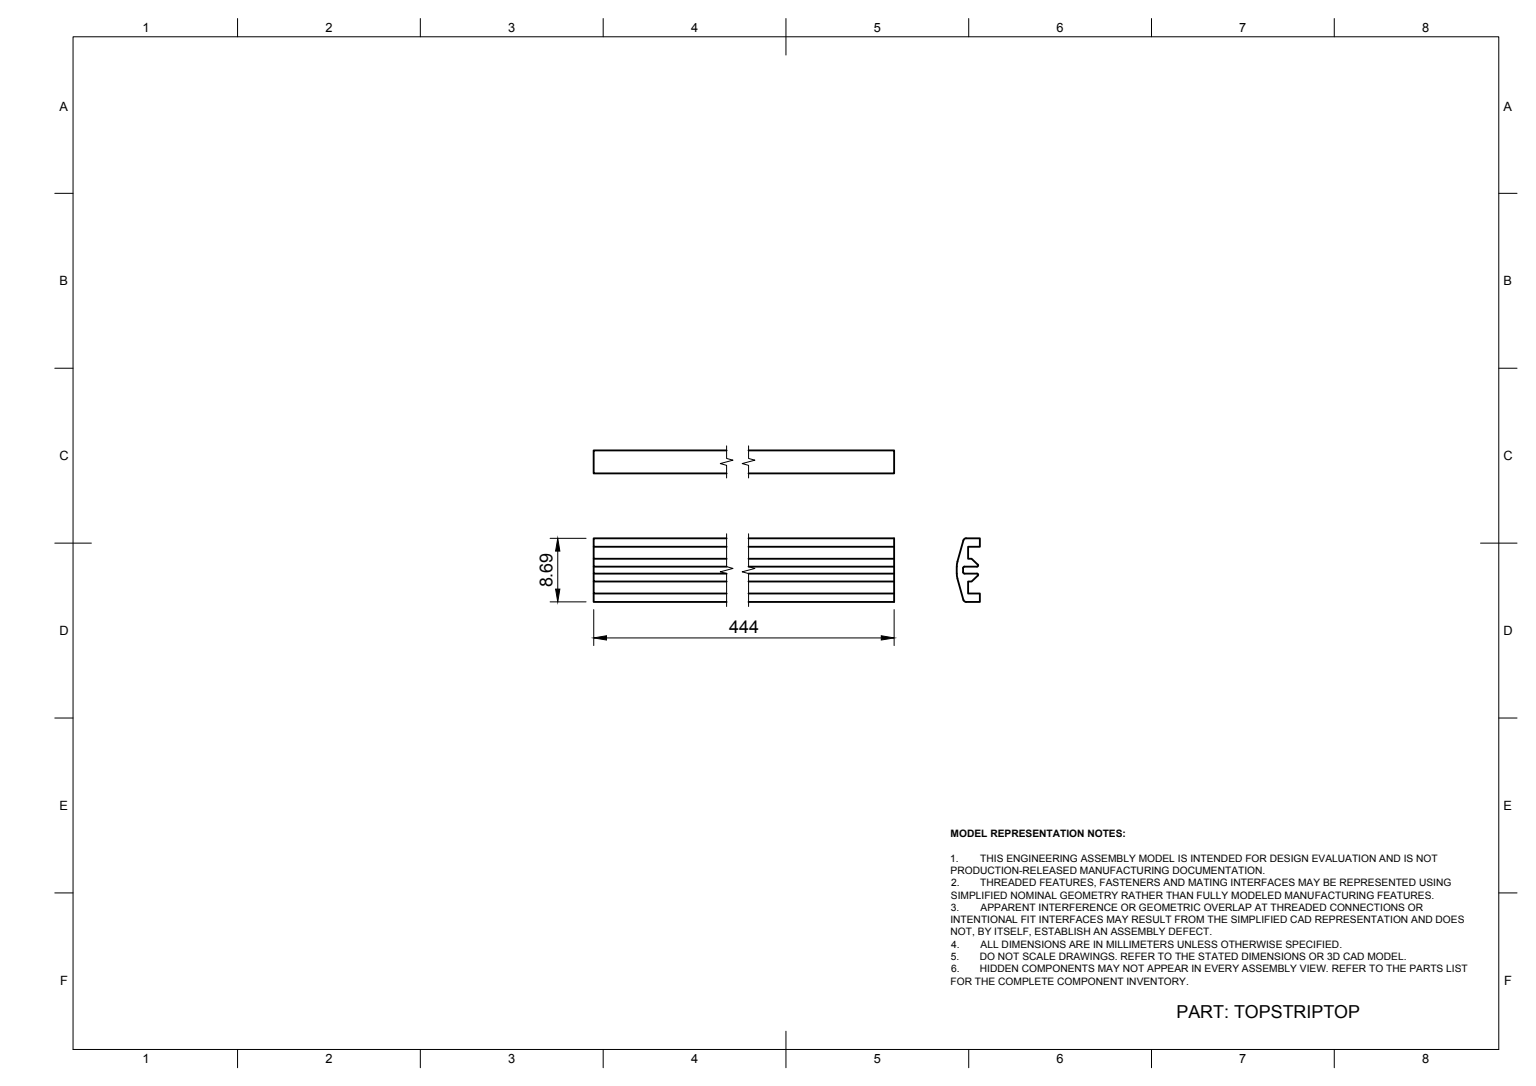
ISO-10303-21;
HEADER;
/* Generated by software containing ST-Developer
 * from STEP Tools, Inc. (www.steptools.com) 
 */

FILE_DESCRIPTION(
/* description */ (''),
/* implementation_level */ '2;1');

FILE_NAME(
/* name */ 'TopStripTop.step',
/* time_stamp */ '2026-10-05T11:01:41-07:00',
/* author */ (''),
/* organization */ (''),
/* preprocessor_version */ 'ST-DEVELOPER v20.2',
/* originating_system */ 'Autodesk Translation Framework v15.15.0.0',
/* authorisation */ '');

FILE_SCHEMA (('AUTOMOTIVE_DESIGN { 1 0 10303 214 3 1 1 }'));
ENDSEC;

DATA;
#10=MECHANICAL_DESIGN_GEOMETRIC_PRESENTATION_REPRESENTATION('',(#2138),#215609);
#2120=SHAPE_REPRESENTATION_RELATIONSHIP('SRR','None',#215645,#2129);
#2129=ADVANCED_BREP_SHAPE_REPRESENTATION('',(#2147),#215601);
#2138=STYLED_ITEM('',(#215698),#2147);
#2147=MANIFOLD_SOLID_BREP('Body1',#28081);
#2165=CYLINDRICAL_SURFACE('',#28237,0.203000000000002);
#2166=CYLINDRICAL_SURFACE('',#28240,0.203000000000002);
#2167=CYLINDRICAL_SURFACE('',#28243,0.159);
#2168=CYLINDRICAL_SURFACE('',#28251,0.381);
#2169=CYLINDRICAL_SURFACE('',#28254,2.54);
#2170=CYLINDRICAL_SURFACE('',#28257,2.54);
#2171=CYLINDRICAL_SURFACE('',#28260,0.381);
#2172=CYLINDRICAL_SURFACE('',#28268,0.159);
#2991=FACE_OUTER_BOUND('',#4304,.T.);
#2992=FACE_OUTER_BOUND('',#4305,.T.);
#2993=FACE_OUTER_BOUND('',#4306,.T.);
#2994=FACE_OUTER_BOUND('',#4307,.T.);
#2995=FACE_OUTER_BOUND('',#4308,.T.);
#2996=FACE_OUTER_BOUND('',#4309,.T.);
#2997=FACE_OUTER_BOUND('',#4310,.T.);
#2998=FACE_OUTER_BOUND('',#4311,.T.);
#2999=FACE_OUTER_BOUND('',#4312,.T.);
#3000=FACE_OUTER_BOUND('',#4313,.T.);
#3001=FACE_OUTER_BOUND('',#4314,.T.);
#3002=FACE_OUTER_BOUND('',#4315,.T.);
#3003=FACE_OUTER_BOUND('',#4316,.T.);
#3004=FACE_OUTER_BOUND('',#4317,.T.);
#3005=FACE_OUTER_BOUND('',#4318,.T.);
#3006=FACE_OUTER_BOUND('',#4319,.T.);
#3007=FACE_OUTER_BOUND('',#4320,.T.);
#3008=FACE_OUTER_BOUND('',#4321,.T.);
#3009=FACE_OUTER_BOUND('',#4322,.T.);
#3010=FACE_OUTER_BOUND('',#4323,.T.);
#3011=FACE_OUTER_BOUND('',#4324,.T.);
#3012=FACE_OUTER_BOUND('',#4325,.T.);
#3013=FACE_OUTER_BOUND('',#4326,.T.);
#3014=FACE_OUTER_BOUND('',#4327,.T.);
#3015=FACE_OUTER_BOUND('',#4328,.T.);
#3016=FACE_OUTER_BOUND('',#4329,.T.);
#3017=FACE_OUTER_BOUND('',#4330,.T.);
#3018=FACE_OUTER_BOUND('',#4331,.T.);
#4304=EDGE_LOOP('',(#17679,#17680,#17681,#17682,#17683,#17684,#17685,#17686,
#17687,#17688,#17689,#17690,#17691,#17692,#17693,#17694,#17695,#17696,#17697,
#17698,#17699,#17700,#17701,#17702,#17703,#17704));
#4305=EDGE_LOOP('',(#17705,#17706,#17707,#17708));
#4306=EDGE_LOOP('',(#17709,#17710,#17711,#17712));
#4307=EDGE_LOOP('',(#17713,#17714,#17715,#17716));
#4308=EDGE_LOOP('',(#17717,#17718,#17719,#17720));
#4309=EDGE_LOOP('',(#17721,#17722,#17723,#17724));
#4310=EDGE_LOOP('',(#17725,#17726,#17727,#17728));
#4311=EDGE_LOOP('',(#17729,#17730,#17731,#17732));
#4312=EDGE_LOOP('',(#17733,#17734,#17735,#17736));
#4313=EDGE_LOOP('',(#17737,#17738,#17739,#17740));
#4314=EDGE_LOOP('',(#17741,#17742,#17743,#17744));
#4315=EDGE_LOOP('',(#17745,#17746,#17747,#17748));
#4316=EDGE_LOOP('',(#17749,#17750,#17751,#17752));
#4317=EDGE_LOOP('',(#17753,#17754,#17755,#17756));
#4318=EDGE_LOOP('',(#17757,#17758,#17759,#17760));
#4319=EDGE_LOOP('',(#17761,#17762,#17763,#17764));
#4320=EDGE_LOOP('',(#17765,#17766,#17767,#17768));
#4321=EDGE_LOOP('',(#17769,#17770,#17771,#17772));
#4322=EDGE_LOOP('',(#17773,#17774,#17775,#17776));
#4323=EDGE_LOOP('',(#17777,#17778,#17779,#17780));
#4324=EDGE_LOOP('',(#17781,#17782,#17783,#17784));
#4325=EDGE_LOOP('',(#17785,#17786,#17787,#17788));
#4326=EDGE_LOOP('',(#17789,#17790,#17791,#17792));
#4327=EDGE_LOOP('',(#17793,#17794,#17795,#17796));
#4328=EDGE_LOOP('',(#17797,#17798,#17799,#17800));
#4329=EDGE_LOOP('',(#17801,#17802,#17803,#17804));
#4330=EDGE_LOOP('',(#17805,#17806,#17807,#17808));
#4331=EDGE_LOOP('',(#17809,#17810,#17811,#17812,#17813,#17814,#17815,#17816,
#17817,#17818,#17819,#17820,#17821,#17822,#17823,#17824,#17825,#17826,#17827,
#17828,#17829,#17830,#17831,#17832,#17833,#17834));
#5684=CIRCLE('',#28229,0.203000000000002);
#5685=CIRCLE('',#28230,0.203000000000002);
#5686=CIRCLE('',#28231,0.159);
#5687=CIRCLE('',#28232,0.381);
#5688=CIRCLE('',#28233,2.54);
#5689=CIRCLE('',#28234,2.54);
#5690=CIRCLE('',#28235,0.381);
#5691=CIRCLE('',#28236,0.159);
#5692=CIRCLE('',#28238,0.203000000000002);
#5693=CIRCLE('',#28241,0.203000000000002);
#5694=CIRCLE('',#28244,0.159);
#5695=CIRCLE('',#28252,0.381);
#5696=CIRCLE('',#28255,2.54);
#5697=CIRCLE('',#28258,2.54);
#5698=CIRCLE('',#28261,0.381);
#5699=CIRCLE('',#28269,0.159);
#6351=LINE('',#36139,#8196);
#6352=LINE('',#36143,#8197);
#6353=LINE('',#36147,#8198);
#6354=LINE('',#36151,#8199);
#6355=LINE('',#36153,#8200);
#6356=LINE('',#36155,#8201);
#6357=LINE('',#36157,#8202);
#6358=LINE('',#36159,#8203);
#6359=LINE('',#36161,#8204);
#6360=LINE('',#36165,#8205);
#6361=LINE('',#36169,#8206);
#6362=LINE('',#36173,#8207);
#6363=LINE('',#36177,#8208);
#6364=LINE('',#36179,#8209);
#6365=LINE('',#36181,#8210);
#6366=LINE('',#36183,#8211);
#6367=LINE('',#36185,#8212);
#6368=LINE('',#36187,#8213);
#6369=LINE('',#36191,#8214);
#6370=LINE('',#36194,#8215);
#6371=LINE('',#36197,#8216);
#6372=LINE('',#36198,#8217);
#6373=LINE('',#36202,#8218);
#6374=LINE('',#36205,#8219);
#6375=LINE('',#36206,#8220);
#6376=LINE('',#36210,#8221);
#6377=LINE('',#36213,#8222);
#6378=LINE('',#36214,#8223);
#6379=LINE('',#36217,#8224);
#6380=LINE('',#36218,#8225);
#6381=LINE('',#36221,#8226);
#6382=LINE('',#36222,#8227);
#6383=LINE('',#36225,#8228);
#6384=LINE('',#36226,#8229);
#6385=LINE('',#36229,#8230);
#6386=LINE('',#36230,#8231);
#6387=LINE('',#36233,#8232);
#6388=LINE('',#36234,#8233);
#6389=LINE('',#36238,#8234);
#6390=LINE('',#36241,#8235);
#6391=LINE('',#36242,#8236);
#6392=LINE('',#36246,#8237);
#6393=LINE('',#36249,#8238);
#6394=LINE('',#36250,#8239);
#6395=LINE('',#36254,#8240);
#6396=LINE('',#36257,#8241);
#6397=LINE('',#36258,#8242);
#6398=LINE('',#36262,#8243);
#6399=LINE('',#36265,#8244);
#6400=LINE('',#36266,#8245);
#6401=LINE('',#36269,#8246);
#6402=LINE('',#36270,#8247);
#6403=LINE('',#36273,#8248);
#6404=LINE('',#36274,#8249);
#6405=LINE('',#36277,#8250);
#6406=LINE('',#36278,#8251);
#6407=LINE('',#36281,#8252);
#6408=LINE('',#36282,#8253);
#6409=LINE('',#36285,#8254);
#6410=LINE('',#36286,#8255);
#6411=LINE('',#36290,#8256);
#6412=LINE('',#36292,#8257);
#8196=VECTOR('',#30321,10.);
#8197=VECTOR('',#30324,10.);
#8198=VECTOR('',#30327,10.);
#8199=VECTOR('',#30330,10.);
#8200=VECTOR('',#30331,10.);
#8201=VECTOR('',#30332,10.);
#8202=VECTOR('',#30333,10.);
#8203=VECTOR('',#30334,10.);
#8204=VECTOR('',#30335,10.);
#8205=VECTOR('',#30338,10.);
#8206=VECTOR('',#30341,10.);
#8207=VECTOR('',#30344,10.);
#8208=VECTOR('',#30347,10.);
#8209=VECTOR('',#30348,10.);
#8210=VECTOR('',#30349,10.);
#8211=VECTOR('',#30350,10.);
#8212=VECTOR('',#30351,10.);
#8213=VECTOR('',#30352,10.);
#8214=VECTOR('',#30357,10.);
#8215=VECTOR('',#30360,10.);
#8216=VECTOR('',#30363,10.);
#8217=VECTOR('',#30364,10.);
#8218=VECTOR('',#30369,10.);
#8219=VECTOR('',#30372,10.);
#8220=VECTOR('',#30373,10.);
#8221=VECTOR('',#30378,10.);
#8222=VECTOR('',#30381,10.);
#8223=VECTOR('',#30382,10.);
#8224=VECTOR('',#30385,10.);
#8225=VECTOR('',#30386,10.);
#8226=VECTOR('',#30389,10.);
#8227=VECTOR('',#30390,10.);
#8228=VECTOR('',#30393,10.);
#8229=VECTOR('',#30394,10.);
#8230=VECTOR('',#30397,10.);
#8231=VECTOR('',#30398,10.);
#8232=VECTOR('',#30401,10.);
#8233=VECTOR('',#30402,10.);
#8234=VECTOR('',#30407,10.);
#8235=VECTOR('',#30410,10.);
#8236=VECTOR('',#30411,10.);
#8237=VECTOR('',#30416,10.);
#8238=VECTOR('',#30419,10.);
#8239=VECTOR('',#30420,10.);
#8240=VECTOR('',#30425,10.);
#8241=VECTOR('',#30428,10.);
#8242=VECTOR('',#30429,10.);
#8243=VECTOR('',#30434,10.);
#8244=VECTOR('',#30437,10.);
#8245=VECTOR('',#30438,10.);
#8246=VECTOR('',#30441,10.);
#8247=VECTOR('',#30442,10.);
#8248=VECTOR('',#30445,10.);
#8249=VECTOR('',#30446,10.);
#8250=VECTOR('',#30449,10.);
#8251=VECTOR('',#30450,10.);
#8252=VECTOR('',#30453,10.);
#8253=VECTOR('',#30454,10.);
#8254=VECTOR('',#30457,10.);
#8255=VECTOR('',#30458,10.);
#8256=VECTOR('',#30463,10.);
#8257=VECTOR('',#30466,10.);
#10036=VERTEX_POINT('',#36137);
#10037=VERTEX_POINT('',#36138);
#10038=VERTEX_POINT('',#36140);
#10039=VERTEX_POINT('',#36142);
#10040=VERTEX_POINT('',#36144);
#10041=VERTEX_POINT('',#36146);
#10042=VERTEX_POINT('',#36148);
#10043=VERTEX_POINT('',#36150);
#10044=VERTEX_POINT('',#36152);
#10045=VERTEX_POINT('',#36154);
#10046=VERTEX_POINT('',#36156);
#10047=VERTEX_POINT('',#36158);
#10048=VERTEX_POINT('',#36160);
#10049=VERTEX_POINT('',#36162);
#10050=VERTEX_POINT('',#36164);
#10051=VERTEX_POINT('',#36166);
#10052=VERTEX_POINT('',#36168);
#10053=VERTEX_POINT('',#36170);
#10054=VERTEX_POINT('',#36172);
#10055=VERTEX_POINT('',#36174);
#10056=VERTEX_POINT('',#36176);
#10057=VERTEX_POINT('',#36178);
#10058=VERTEX_POINT('',#36180);
#10059=VERTEX_POINT('',#36182);
#10060=VERTEX_POINT('',#36184);
#10061=VERTEX_POINT('',#36186);
#10062=VERTEX_POINT('',#36190);
#10063=VERTEX_POINT('',#36192);
#10064=VERTEX_POINT('',#36196);
#10065=VERTEX_POINT('',#36200);
#10066=VERTEX_POINT('',#36204);
#10067=VERTEX_POINT('',#36208);
#10068=VERTEX_POINT('',#36212);
#10069=VERTEX_POINT('',#36216);
#10070=VERTEX_POINT('',#36220);
#10071=VERTEX_POINT('',#36224);
#10072=VERTEX_POINT('',#36228);
#10073=VERTEX_POINT('',#36232);
#10074=VERTEX_POINT('',#36236);
#10075=VERTEX_POINT('',#36240);
#10076=VERTEX_POINT('',#36244);
#10077=VERTEX_POINT('',#36248);
#10078=VERTEX_POINT('',#36252);
#10079=VERTEX_POINT('',#36256);
#10080=VERTEX_POINT('',#36260);
#10081=VERTEX_POINT('',#36264);
#10082=VERTEX_POINT('',#36268);
#10083=VERTEX_POINT('',#36272);
#10084=VERTEX_POINT('',#36276);
#10085=VERTEX_POINT('',#36280);
#10086=VERTEX_POINT('',#36284);
#10087=VERTEX_POINT('',#36288);
#13201=EDGE_CURVE('',#10036,#10037,#6351,.T.);
#13202=EDGE_CURVE('',#10037,#10038,#5684,.T.);
#13203=EDGE_CURVE('',#10038,#10039,#6352,.T.);
#13204=EDGE_CURVE('',#10039,#10040,#5685,.T.);
#13205=EDGE_CURVE('',#10040,#10041,#6353,.T.);
#13206=EDGE_CURVE('',#10041,#10042,#5686,.T.);
#13207=EDGE_CURVE('',#10042,#10043,#6354,.T.);
#13208=EDGE_CURVE('',#10043,#10044,#6355,.T.);
#13209=EDGE_CURVE('',#10044,#10045,#6356,.T.);
#13210=EDGE_CURVE('',#10045,#10046,#6357,.T.);
#13211=EDGE_CURVE('',#10046,#10047,#6358,.T.);
#13212=EDGE_CURVE('',#10047,#10048,#6359,.T.);
#13213=EDGE_CURVE('',#10048,#10049,#5687,.T.);
#13214=EDGE_CURVE('',#10049,#10050,#6360,.T.);
#13215=EDGE_CURVE('',#10050,#10051,#5688,.T.);
#13216=EDGE_CURVE('',#10051,#10052,#6361,.T.);
#13217=EDGE_CURVE('',#10052,#10053,#5689,.T.);
#13218=EDGE_CURVE('',#10053,#10054,#6362,.T.);
#13219=EDGE_CURVE('',#10054,#10055,#5690,.T.);
#13220=EDGE_CURVE('',#10055,#10056,#6363,.T.);
#13221=EDGE_CURVE('',#10056,#10057,#6364,.T.);
#13222=EDGE_CURVE('',#10057,#10058,#6365,.T.);
#13223=EDGE_CURVE('',#10058,#10059,#6366,.T.);
#13224=EDGE_CURVE('',#10059,#10060,#6367,.T.);
#13225=EDGE_CURVE('',#10060,#10061,#6368,.T.);
#13226=EDGE_CURVE('',#10061,#10036,#5691,.T.);
#13227=EDGE_CURVE('',#10062,#10037,#6369,.T.);
#13228=EDGE_CURVE('',#10063,#10062,#5692,.T.);
#13229=EDGE_CURVE('',#10038,#10063,#6370,.T.);
#13230=EDGE_CURVE('',#10064,#10063,#6371,.T.);
#13231=EDGE_CURVE('',#10039,#10064,#6372,.T.);
#13232=EDGE_CURVE('',#10065,#10064,#5693,.T.);
#13233=EDGE_CURVE('',#10040,#10065,#6373,.T.);
#13234=EDGE_CURVE('',#10066,#10065,#6374,.T.);
#13235=EDGE_CURVE('',#10041,#10066,#6375,.T.);
#13236=EDGE_CURVE('',#10067,#10066,#5694,.T.);
#13237=EDGE_CURVE('',#10042,#10067,#6376,.T.);
#13238=EDGE_CURVE('',#10068,#10067,#6377,.T.);
#13239=EDGE_CURVE('',#10043,#10068,#6378,.T.);
#13240=EDGE_CURVE('',#10069,#10068,#6379,.T.);
#13241=EDGE_CURVE('',#10044,#10069,#6380,.T.);
#13242=EDGE_CURVE('',#10070,#10069,#6381,.T.);
#13243=EDGE_CURVE('',#10045,#10070,#6382,.T.);
#13244=EDGE_CURVE('',#10071,#10070,#6383,.T.);
#13245=EDGE_CURVE('',#10046,#10071,#6384,.T.);
#13246=EDGE_CURVE('',#10072,#10071,#6385,.T.);
#13247=EDGE_CURVE('',#10047,#10072,#6386,.T.);
#13248=EDGE_CURVE('',#10073,#10072,#6387,.T.);
#13249=EDGE_CURVE('',#10048,#10073,#6388,.T.);
#13250=EDGE_CURVE('',#10074,#10073,#5695,.T.);
#13251=EDGE_CURVE('',#10049,#10074,#6389,.T.);
#13252=EDGE_CURVE('',#10075,#10074,#6390,.T.);
#13253=EDGE_CURVE('',#10050,#10075,#6391,.T.);
#13254=EDGE_CURVE('',#10076,#10075,#5696,.T.);
#13255=EDGE_CURVE('',#10051,#10076,#6392,.T.);
#13256=EDGE_CURVE('',#10077,#10076,#6393,.T.);
#13257=EDGE_CURVE('',#10052,#10077,#6394,.T.);
#13258=EDGE_CURVE('',#10078,#10077,#5697,.T.);
#13259=EDGE_CURVE('',#10053,#10078,#6395,.T.);
#13260=EDGE_CURVE('',#10079,#10078,#6396,.T.);
#13261=EDGE_CURVE('',#10054,#10079,#6397,.T.);
#13262=EDGE_CURVE('',#10080,#10079,#5698,.T.);
#13263=EDGE_CURVE('',#10055,#10080,#6398,.T.);
#13264=EDGE_CURVE('',#10081,#10080,#6399,.T.);
#13265=EDGE_CURVE('',#10056,#10081,#6400,.T.);
#13266=EDGE_CURVE('',#10082,#10081,#6401,.T.);
#13267=EDGE_CURVE('',#10057,#10082,#6402,.T.);
#13268=EDGE_CURVE('',#10083,#10082,#6403,.T.);
#13269=EDGE_CURVE('',#10058,#10083,#6404,.T.);
#13270=EDGE_CURVE('',#10084,#10083,#6405,.T.);
#13271=EDGE_CURVE('',#10059,#10084,#6406,.T.);
#13272=EDGE_CURVE('',#10085,#10084,#6407,.T.);
#13273=EDGE_CURVE('',#10060,#10085,#6408,.T.);
#13274=EDGE_CURVE('',#10086,#10085,#6409,.T.);
#13275=EDGE_CURVE('',#10061,#10086,#6410,.T.);
#13276=EDGE_CURVE('',#10087,#10086,#5699,.T.);
#13277=EDGE_CURVE('',#10036,#10087,#6411,.T.);
#13278=EDGE_CURVE('',#10062,#10087,#6412,.T.);
#17679=ORIENTED_EDGE('',*,*,#13201,.T.);
#17680=ORIENTED_EDGE('',*,*,#13202,.T.);
#17681=ORIENTED_EDGE('',*,*,#13203,.T.);
#17682=ORIENTED_EDGE('',*,*,#13204,.T.);
#17683=ORIENTED_EDGE('',*,*,#13205,.T.);
#17684=ORIENTED_EDGE('',*,*,#13206,.T.);
#17685=ORIENTED_EDGE('',*,*,#13207,.T.);
#17686=ORIENTED_EDGE('',*,*,#13208,.T.);
#17687=ORIENTED_EDGE('',*,*,#13209,.T.);
#17688=ORIENTED_EDGE('',*,*,#13210,.T.);
#17689=ORIENTED_EDGE('',*,*,#13211,.T.);
#17690=ORIENTED_EDGE('',*,*,#13212,.T.);
#17691=ORIENTED_EDGE('',*,*,#13213,.T.);
#17692=ORIENTED_EDGE('',*,*,#13214,.T.);
#17693=ORIENTED_EDGE('',*,*,#13215,.T.);
#17694=ORIENTED_EDGE('',*,*,#13216,.T.);
#17695=ORIENTED_EDGE('',*,*,#13217,.T.);
#17696=ORIENTED_EDGE('',*,*,#13218,.T.);
#17697=ORIENTED_EDGE('',*,*,#13219,.T.);
#17698=ORIENTED_EDGE('',*,*,#13220,.T.);
#17699=ORIENTED_EDGE('',*,*,#13221,.T.);
#17700=ORIENTED_EDGE('',*,*,#13222,.T.);
#17701=ORIENTED_EDGE('',*,*,#13223,.T.);
#17702=ORIENTED_EDGE('',*,*,#13224,.T.);
#17703=ORIENTED_EDGE('',*,*,#13225,.T.);
#17704=ORIENTED_EDGE('',*,*,#13226,.T.);
#17705=ORIENTED_EDGE('',*,*,#13227,.F.);
#17706=ORIENTED_EDGE('',*,*,#13228,.F.);
#17707=ORIENTED_EDGE('',*,*,#13229,.F.);
#17708=ORIENTED_EDGE('',*,*,#13202,.F.);
#17709=ORIENTED_EDGE('',*,*,#13229,.T.);
#17710=ORIENTED_EDGE('',*,*,#13230,.F.);
#17711=ORIENTED_EDGE('',*,*,#13231,.F.);
#17712=ORIENTED_EDGE('',*,*,#13203,.F.);
#17713=ORIENTED_EDGE('',*,*,#13231,.T.);
#17714=ORIENTED_EDGE('',*,*,#13232,.F.);
#17715=ORIENTED_EDGE('',*,*,#13233,.F.);
#17716=ORIENTED_EDGE('',*,*,#13204,.F.);
#17717=ORIENTED_EDGE('',*,*,#13233,.T.);
#17718=ORIENTED_EDGE('',*,*,#13234,.F.);
#17719=ORIENTED_EDGE('',*,*,#13235,.F.);
#17720=ORIENTED_EDGE('',*,*,#13205,.F.);
#17721=ORIENTED_EDGE('',*,*,#13235,.T.);
#17722=ORIENTED_EDGE('',*,*,#13236,.F.);
#17723=ORIENTED_EDGE('',*,*,#13237,.F.);
#17724=ORIENTED_EDGE('',*,*,#13206,.F.);
#17725=ORIENTED_EDGE('',*,*,#13237,.T.);
#17726=ORIENTED_EDGE('',*,*,#13238,.F.);
#17727=ORIENTED_EDGE('',*,*,#13239,.F.);
#17728=ORIENTED_EDGE('',*,*,#13207,.F.);
#17729=ORIENTED_EDGE('',*,*,#13239,.T.);
#17730=ORIENTED_EDGE('',*,*,#13240,.F.);
#17731=ORIENTED_EDGE('',*,*,#13241,.F.);
#17732=ORIENTED_EDGE('',*,*,#13208,.F.);
#17733=ORIENTED_EDGE('',*,*,#13241,.T.);
#17734=ORIENTED_EDGE('',*,*,#13242,.F.);
#17735=ORIENTED_EDGE('',*,*,#13243,.F.);
#17736=ORIENTED_EDGE('',*,*,#13209,.F.);
#17737=ORIENTED_EDGE('',*,*,#13243,.T.);
#17738=ORIENTED_EDGE('',*,*,#13244,.F.);
#17739=ORIENTED_EDGE('',*,*,#13245,.F.);
#17740=ORIENTED_EDGE('',*,*,#13210,.F.);
#17741=ORIENTED_EDGE('',*,*,#13245,.T.);
#17742=ORIENTED_EDGE('',*,*,#13246,.F.);
#17743=ORIENTED_EDGE('',*,*,#13247,.F.);
#17744=ORIENTED_EDGE('',*,*,#13211,.F.);
#17745=ORIENTED_EDGE('',*,*,#13247,.T.);
#17746=ORIENTED_EDGE('',*,*,#13248,.F.);
#17747=ORIENTED_EDGE('',*,*,#13249,.F.);
#17748=ORIENTED_EDGE('',*,*,#13212,.F.);
#17749=ORIENTED_EDGE('',*,*,#13249,.T.);
#17750=ORIENTED_EDGE('',*,*,#13250,.F.);
#17751=ORIENTED_EDGE('',*,*,#13251,.F.);
#17752=ORIENTED_EDGE('',*,*,#13213,.F.);
#17753=ORIENTED_EDGE('',*,*,#13251,.T.);
#17754=ORIENTED_EDGE('',*,*,#13252,.F.);
#17755=ORIENTED_EDGE('',*,*,#13253,.F.);
#17756=ORIENTED_EDGE('',*,*,#13214,.F.);
#17757=ORIENTED_EDGE('',*,*,#13253,.T.);
#17758=ORIENTED_EDGE('',*,*,#13254,.F.);
#17759=ORIENTED_EDGE('',*,*,#13255,.F.);
#17760=ORIENTED_EDGE('',*,*,#13215,.F.);
#17761=ORIENTED_EDGE('',*,*,#13255,.T.);
#17762=ORIENTED_EDGE('',*,*,#13256,.F.);
#17763=ORIENTED_EDGE('',*,*,#13257,.F.);
#17764=ORIENTED_EDGE('',*,*,#13216,.F.);
#17765=ORIENTED_EDGE('',*,*,#13257,.T.);
#17766=ORIENTED_EDGE('',*,*,#13258,.F.);
#17767=ORIENTED_EDGE('',*,*,#13259,.F.);
#17768=ORIENTED_EDGE('',*,*,#13217,.F.);
#17769=ORIENTED_EDGE('',*,*,#13259,.T.);
#17770=ORIENTED_EDGE('',*,*,#13260,.F.);
#17771=ORIENTED_EDGE('',*,*,#13261,.F.);
#17772=ORIENTED_EDGE('',*,*,#13218,.F.);
#17773=ORIENTED_EDGE('',*,*,#13261,.T.);
#17774=ORIENTED_EDGE('',*,*,#13262,.F.);
#17775=ORIENTED_EDGE('',*,*,#13263,.F.);
#17776=ORIENTED_EDGE('',*,*,#13219,.F.);
#17777=ORIENTED_EDGE('',*,*,#13263,.T.);
#17778=ORIENTED_EDGE('',*,*,#13264,.F.);
#17779=ORIENTED_EDGE('',*,*,#13265,.F.);
#17780=ORIENTED_EDGE('',*,*,#13220,.F.);
#17781=ORIENTED_EDGE('',*,*,#13265,.T.);
#17782=ORIENTED_EDGE('',*,*,#13266,.F.);
#17783=ORIENTED_EDGE('',*,*,#13267,.F.);
#17784=ORIENTED_EDGE('',*,*,#13221,.F.);
#17785=ORIENTED_EDGE('',*,*,#13267,.T.);
#17786=ORIENTED_EDGE('',*,*,#13268,.F.);
#17787=ORIENTED_EDGE('',*,*,#13269,.F.);
#17788=ORIENTED_EDGE('',*,*,#13222,.F.);
#17789=ORIENTED_EDGE('',*,*,#13269,.T.);
#17790=ORIENTED_EDGE('',*,*,#13270,.F.);
#17791=ORIENTED_EDGE('',*,*,#13271,.F.);
#17792=ORIENTED_EDGE('',*,*,#13223,.F.);
#17793=ORIENTED_EDGE('',*,*,#13271,.T.);
#17794=ORIENTED_EDGE('',*,*,#13272,.F.);
#17795=ORIENTED_EDGE('',*,*,#13273,.F.);
#17796=ORIENTED_EDGE('',*,*,#13224,.F.);
#17797=ORIENTED_EDGE('',*,*,#13273,.T.);
#17798=ORIENTED_EDGE('',*,*,#13274,.F.);
#17799=ORIENTED_EDGE('',*,*,#13275,.F.);
#17800=ORIENTED_EDGE('',*,*,#13225,.F.);
#17801=ORIENTED_EDGE('',*,*,#13275,.T.);
#17802=ORIENTED_EDGE('',*,*,#13276,.F.);
#17803=ORIENTED_EDGE('',*,*,#13277,.F.);
#17804=ORIENTED_EDGE('',*,*,#13226,.F.);
#17805=ORIENTED_EDGE('',*,*,#13277,.T.);
#17806=ORIENTED_EDGE('',*,*,#13278,.F.);
#17807=ORIENTED_EDGE('',*,*,#13227,.T.);
#17808=ORIENTED_EDGE('',*,*,#13201,.F.);
#17809=ORIENTED_EDGE('',*,*,#13278,.T.);
#17810=ORIENTED_EDGE('',*,*,#13276,.T.);
#17811=ORIENTED_EDGE('',*,*,#13274,.T.);
#17812=ORIENTED_EDGE('',*,*,#13272,.T.);
#17813=ORIENTED_EDGE('',*,*,#13270,.T.);
#17814=ORIENTED_EDGE('',*,*,#13268,.T.);
#17815=ORIENTED_EDGE('',*,*,#13266,.T.);
#17816=ORIENTED_EDGE('',*,*,#13264,.T.);
#17817=ORIENTED_EDGE('',*,*,#13262,.T.);
#17818=ORIENTED_EDGE('',*,*,#13260,.T.);
#17819=ORIENTED_EDGE('',*,*,#13258,.T.);
#17820=ORIENTED_EDGE('',*,*,#13256,.T.);
#17821=ORIENTED_EDGE('',*,*,#13254,.T.);
#17822=ORIENTED_EDGE('',*,*,#13252,.T.);
#17823=ORIENTED_EDGE('',*,*,#13250,.T.);
#17824=ORIENTED_EDGE('',*,*,#13248,.T.);
#17825=ORIENTED_EDGE('',*,*,#13246,.T.);
#17826=ORIENTED_EDGE('',*,*,#13244,.T.);
#17827=ORIENTED_EDGE('',*,*,#13242,.T.);
#17828=ORIENTED_EDGE('',*,*,#13240,.T.);
#17829=ORIENTED_EDGE('',*,*,#13238,.T.);
#17830=ORIENTED_EDGE('',*,*,#13236,.T.);
#17831=ORIENTED_EDGE('',*,*,#13234,.T.);
#17832=ORIENTED_EDGE('',*,*,#13232,.T.);
#17833=ORIENTED_EDGE('',*,*,#13230,.T.);
#17834=ORIENTED_EDGE('',*,*,#13228,.T.);
#26352=PLANE('',#28228);
#26353=PLANE('',#28239);
#26354=PLANE('',#28242);
#26355=PLANE('',#28245);
#26356=PLANE('',#28246);
#26357=PLANE('',#28247);
#26358=PLANE('',#28248);
#26359=PLANE('',#28249);
#26360=PLANE('',#28250);
#26361=PLANE('',#28253);
#26362=PLANE('',#28256);
#26363=PLANE('',#28259);
#26364=PLANE('',#28262);
#26365=PLANE('',#28263);
#26366=PLANE('',#28264);
#26367=PLANE('',#28265);
#26368=PLANE('',#28266);
#26369=PLANE('',#28267);
#26370=PLANE('',#28270);
#26371=PLANE('',#28271);
#26794=ADVANCED_FACE('',(#2991),#26352,.F.);
#26795=ADVANCED_FACE('',(#2992),#2165,.F.);
#26796=ADVANCED_FACE('',(#2993),#26353,.T.);
#26797=ADVANCED_FACE('',(#2994),#2166,.F.);
#26798=ADVANCED_FACE('',(#2995),#26354,.T.);
#26799=ADVANCED_FACE('',(#2996),#2167,.T.);
#26800=ADVANCED_FACE('',(#2997),#26355,.T.);
#26801=ADVANCED_FACE('',(#2998),#26356,.T.);
#26802=ADVANCED_FACE('',(#2999),#26357,.T.);
#26803=ADVANCED_FACE('',(#3000),#26358,.T.);
#26804=ADVANCED_FACE('',(#3001),#26359,.T.);
#26805=ADVANCED_FACE('',(#3002),#26360,.T.);
#26806=ADVANCED_FACE('',(#3003),#2168,.T.);
#26807=ADVANCED_FACE('',(#3004),#26361,.T.);
#26808=ADVANCED_FACE('',(#3005),#2169,.T.);
#26809=ADVANCED_FACE('',(#3006),#26362,.T.);
#26810=ADVANCED_FACE('',(#3007),#2170,.T.);
#26811=ADVANCED_FACE('',(#3008),#26363,.T.);
#26812=ADVANCED_FACE('',(#3009),#2171,.T.);
#26813=ADVANCED_FACE('',(#3010),#26364,.T.);
#26814=ADVANCED_FACE('',(#3011),#26365,.T.);
#26815=ADVANCED_FACE('',(#3012),#26366,.T.);
#26816=ADVANCED_FACE('',(#3013),#26367,.T.);
#26817=ADVANCED_FACE('',(#3014),#26368,.T.);
#26818=ADVANCED_FACE('',(#3015),#26369,.T.);
#26819=ADVANCED_FACE('',(#3016),#2172,.T.);
#26820=ADVANCED_FACE('',(#3017),#26370,.T.);
#26821=ADVANCED_FACE('',(#3018),#26371,.T.);
#28081=CLOSED_SHELL('',(#26794,#26795,#26796,#26797,#26798,#26799,#26800,
#26801,#26802,#26803,#26804,#26805,#26806,#26807,#26808,#26809,#26810,#26811,
#26812,#26813,#26814,#26815,#26816,#26817,#26818,#26819,#26820,#26821));
#28227=AXIS2_PLACEMENT_3D('',#36135,#30317,#30318);
#28228=AXIS2_PLACEMENT_3D('',#36136,#30319,#30320);
#28229=AXIS2_PLACEMENT_3D('',#36141,#30322,#30323);
#28230=AXIS2_PLACEMENT_3D('',#36145,#30325,#30326);
#28231=AXIS2_PLACEMENT_3D('',#36149,#30328,#30329);
#28232=AXIS2_PLACEMENT_3D('',#36163,#30336,#30337);
#28233=AXIS2_PLACEMENT_3D('',#36167,#30339,#30340);
#28234=AXIS2_PLACEMENT_3D('',#36171,#30342,#30343);
#28235=AXIS2_PLACEMENT_3D('',#36175,#30345,#30346);
#28236=AXIS2_PLACEMENT_3D('',#36188,#30353,#30354);
#28237=AXIS2_PLACEMENT_3D('',#36189,#30355,#30356);
#28238=AXIS2_PLACEMENT_3D('',#36193,#30358,#30359);
#28239=AXIS2_PLACEMENT_3D('',#36195,#30361,#30362);
#28240=AXIS2_PLACEMENT_3D('',#36199,#30365,#30366);
#28241=AXIS2_PLACEMENT_3D('',#36201,#30367,#30368);
#28242=AXIS2_PLACEMENT_3D('',#36203,#30370,#30371);
#28243=AXIS2_PLACEMENT_3D('',#36207,#30374,#30375);
#28244=AXIS2_PLACEMENT_3D('',#36209,#30376,#30377);
#28245=AXIS2_PLACEMENT_3D('',#36211,#30379,#30380);
#28246=AXIS2_PLACEMENT_3D('',#36215,#30383,#30384);
#28247=AXIS2_PLACEMENT_3D('',#36219,#30387,#30388);
#28248=AXIS2_PLACEMENT_3D('',#36223,#30391,#30392);
#28249=AXIS2_PLACEMENT_3D('',#36227,#30395,#30396);
#28250=AXIS2_PLACEMENT_3D('',#36231,#30399,#30400);
#28251=AXIS2_PLACEMENT_3D('',#36235,#30403,#30404);
#28252=AXIS2_PLACEMENT_3D('',#36237,#30405,#30406);
#28253=AXIS2_PLACEMENT_3D('',#36239,#30408,#30409);
#28254=AXIS2_PLACEMENT_3D('',#36243,#30412,#30413);
#28255=AXIS2_PLACEMENT_3D('',#36245,#30414,#30415);
#28256=AXIS2_PLACEMENT_3D('',#36247,#30417,#30418);
#28257=AXIS2_PLACEMENT_3D('',#36251,#30421,#30422);
#28258=AXIS2_PLACEMENT_3D('',#36253,#30423,#30424);
#28259=AXIS2_PLACEMENT_3D('',#36255,#30426,#30427);
#28260=AXIS2_PLACEMENT_3D('',#36259,#30430,#30431);
#28261=AXIS2_PLACEMENT_3D('',#36261,#30432,#30433);
#28262=AXIS2_PLACEMENT_3D('',#36263,#30435,#30436);
#28263=AXIS2_PLACEMENT_3D('',#36267,#30439,#30440);
#28264=AXIS2_PLACEMENT_3D('',#36271,#30443,#30444);
#28265=AXIS2_PLACEMENT_3D('',#36275,#30447,#30448);
#28266=AXIS2_PLACEMENT_3D('',#36279,#30451,#30452);
#28267=AXIS2_PLACEMENT_3D('',#36283,#30455,#30456);
#28268=AXIS2_PLACEMENT_3D('',#36287,#30459,#30460);
#28269=AXIS2_PLACEMENT_3D('',#36289,#30461,#30462);
#28270=AXIS2_PLACEMENT_3D('',#36291,#30464,#30465);
#28271=AXIS2_PLACEMENT_3D('',#36293,#30467,#30468);
#30317=DIRECTION('axis',(0.,0.,1.));
#30318=DIRECTION('refdir',(1.,0.,0.));
#30319=DIRECTION('center_axis',(0.,0.,1.));
#30320=DIRECTION('ref_axis',(1.,0.,0.));
#30321=DIRECTION('',(0.,1.,0.));
#30322=DIRECTION('center_axis',(0.,0.,1.));
#30323=DIRECTION('ref_axis',(1.,0.,0.));
#30324=DIRECTION('',(-1.,0.,0.));
#30325=DIRECTION('center_axis',(0.,0.,1.));
#30326=DIRECTION('ref_axis',(-1.70908716845004E-15,1.,0.));
#30327=DIRECTION('',(1.88534624677928E-15,-1.,0.));
#30328=DIRECTION('center_axis',(0.,0.,-1.));
#30329=DIRECTION('ref_axis',(-0.721760228098359,-0.69214317387041,0.));
#30330=DIRECTION('',(-0.69214317387041,0.721760228098359,0.));
#30331=DIRECTION('',(-2.36721327212187E-15,1.,0.));
#30332=DIRECTION('',(-1.,-2.72113486427735E-15,0.));
#30333=DIRECTION('',(1.39125692308917E-15,-1.,0.));
#30334=DIRECTION('',(-1.,-1.92080108066636E-15,0.));
#30335=DIRECTION('',(-1.77825364328642E-15,1.,0.));
#30336=DIRECTION('center_axis',(0.,0.,-1.));
#30337=DIRECTION('ref_axis',(-0.268919820615266,0.963162566797658,0.));
#30338=DIRECTION('',(0.963162566797657,0.26891982061527,0.));
#30339=DIRECTION('center_axis',(0.,0.,-1.));
#30340=DIRECTION('ref_axis',(-2.02156751531155E-15,1.,0.));
#30341=DIRECTION('',(1.,0.,0.));
#30342=DIRECTION('center_axis',(0.,0.,-1.));
#30343=DIRECTION('ref_axis',(0.268930215136866,0.963159664534619,0.));
#30344=DIRECTION('',(0.963162566797658,-0.268919820615267,0.));
#30345=DIRECTION('center_axis',(0.,0.,-1.));
#30346=DIRECTION('ref_axis',(1.,0.,0.));
#30347=DIRECTION('',(0.,-1.,0.));
#30348=DIRECTION('',(-1.,0.,0.));
#30349=DIRECTION('',(0.,1.,0.));
#30350=DIRECTION('',(-1.,0.,0.));
#30351=DIRECTION('',(0.,-1.,0.));
#30352=DIRECTION('',(-0.692143173870409,-0.72176022809836,0.));
#30353=DIRECTION('center_axis',(0.,0.,-1.));
#30354=DIRECTION('ref_axis',(-1.,0.,0.));
#30355=DIRECTION('center_axis',(0.,0.,1.));
#30356=DIRECTION('ref_axis',(1.,0.,0.));
#30357=DIRECTION('',(0.,0.,-1.));
#30358=DIRECTION('center_axis',(0.,0.,-1.));
#30359=DIRECTION('ref_axis',(1.,0.,0.));
#30360=DIRECTION('',(0.,0.,1.));
#30361=DIRECTION('center_axis',(0.,-1.,0.));
#30362=DIRECTION('ref_axis',(1.,0.,0.));
#30363=DIRECTION('',(1.,0.,0.));
#30364=DIRECTION('',(0.,0.,1.));
#30365=DIRECTION('center_axis',(0.,0.,1.));
#30366=DIRECTION('ref_axis',(-1.70908716845004E-15,1.,0.));
#30367=DIRECTION('center_axis',(0.,0.,-1.));
#30368=DIRECTION('ref_axis',(-1.70908716845004E-15,1.,0.));
#30369=DIRECTION('',(0.,0.,1.));
#30370=DIRECTION('center_axis',(1.,1.88534624677928E-15,0.));
#30371=DIRECTION('ref_axis',(-1.88534624677928E-15,1.,0.));
#30372=DIRECTION('',(-1.88534624677928E-15,1.,0.));
#30373=DIRECTION('',(0.,0.,1.));
#30374=DIRECTION('center_axis',(0.,0.,1.));
#30375=DIRECTION('ref_axis',(-0.721760228098359,-0.69214317387041,0.));
#30376=DIRECTION('center_axis',(0.,0.,1.));
#30377=DIRECTION('ref_axis',(-0.721760228098359,-0.69214317387041,0.));
#30378=DIRECTION('',(0.,0.,1.));
#30379=DIRECTION('center_axis',(-0.721760228098359,-0.69214317387041,0.));
#30380=DIRECTION('ref_axis',(0.69214317387041,-0.721760228098359,0.));
#30381=DIRECTION('',(0.69214317387041,-0.721760228098359,0.));
#30382=DIRECTION('',(0.,0.,1.));
#30383=DIRECTION('center_axis',(-1.,-2.36721327212187E-15,0.));
#30384=DIRECTION('ref_axis',(2.36721327212187E-15,-1.,0.));
#30385=DIRECTION('',(2.36721327212187E-15,-1.,0.));
#30386=DIRECTION('',(0.,0.,1.));
#30387=DIRECTION('center_axis',(2.72113486427735E-15,-1.,0.));
#30388=DIRECTION('ref_axis',(1.,2.72113486427735E-15,0.));
#30389=DIRECTION('',(1.,2.72113486427735E-15,0.));
#30390=DIRECTION('',(0.,0.,1.));
#30391=DIRECTION('center_axis',(1.,1.39125692308917E-15,0.));
#30392=DIRECTION('ref_axis',(-1.39125692308917E-15,1.,0.));
#30393=DIRECTION('',(-1.39125692308917E-15,1.,0.));
#30394=DIRECTION('',(0.,0.,1.));
#30395=DIRECTION('center_axis',(1.92080108066636E-15,-1.,0.));
#30396=DIRECTION('ref_axis',(1.,1.92080108066636E-15,0.));
#30397=DIRECTION('',(1.,1.92080108066636E-15,0.));
#30398=DIRECTION('',(0.,0.,1.));
#30399=DIRECTION('center_axis',(-1.,-1.77825364328642E-15,0.));
#30400=DIRECTION('ref_axis',(1.77825364328642E-15,-1.,0.));
#30401=DIRECTION('',(1.77825364328642E-15,-1.,0.));
#30402=DIRECTION('',(0.,0.,1.));
#30403=DIRECTION('center_axis',(0.,0.,1.));
#30404=DIRECTION('ref_axis',(-0.268919820615266,0.963162566797658,0.));
#30405=DIRECTION('center_axis',(0.,0.,1.));
#30406=DIRECTION('ref_axis',(-0.268919820615266,0.963162566797658,0.));
#30407=DIRECTION('',(0.,0.,1.));
#30408=DIRECTION('center_axis',(-0.26891982061527,0.963162566797657,0.));
#30409=DIRECTION('ref_axis',(-0.963162566797657,-0.26891982061527,0.));
#30410=DIRECTION('',(-0.963162566797657,-0.26891982061527,0.));
#30411=DIRECTION('',(0.,0.,1.));
#30412=DIRECTION('center_axis',(0.,0.,1.));
#30413=DIRECTION('ref_axis',(-2.02156751531155E-15,1.,0.));
#30414=DIRECTION('center_axis',(0.,0.,1.));
#30415=DIRECTION('ref_axis',(-2.02156751531155E-15,1.,0.));
#30416=DIRECTION('',(0.,0.,1.));
#30417=DIRECTION('center_axis',(0.,1.,0.));
#30418=DIRECTION('ref_axis',(-1.,0.,0.));
#30419=DIRECTION('',(-1.,0.,0.));
#30420=DIRECTION('',(0.,0.,1.));
#30421=DIRECTION('center_axis',(0.,0.,1.));
#30422=DIRECTION('ref_axis',(0.268930215136866,0.963159664534619,0.));
#30423=DIRECTION('center_axis',(0.,0.,1.));
#30424=DIRECTION('ref_axis',(0.268930215136866,0.963159664534619,0.));
#30425=DIRECTION('',(0.,0.,1.));
#30426=DIRECTION('center_axis',(0.268919820615267,0.963162566797658,0.));
#30427=DIRECTION('ref_axis',(-0.963162566797658,0.268919820615267,0.));
#30428=DIRECTION('',(-0.963162566797658,0.268919820615267,0.));
#30429=DIRECTION('',(0.,0.,1.));
#30430=DIRECTION('center_axis',(0.,0.,1.));
#30431=DIRECTION('ref_axis',(1.,0.,0.));
#30432=DIRECTION('center_axis',(0.,0.,1.));
#30433=DIRECTION('ref_axis',(1.,0.,0.));
#30434=DIRECTION('',(0.,0.,1.));
#30435=DIRECTION('center_axis',(1.,0.,0.));
#30436=DIRECTION('ref_axis',(0.,1.,0.));
#30437=DIRECTION('',(0.,1.,0.));
#30438=DIRECTION('',(0.,0.,1.));
#30439=DIRECTION('center_axis',(0.,-1.,0.));
#30440=DIRECTION('ref_axis',(1.,0.,0.));
#30441=DIRECTION('',(1.,0.,0.));
#30442=DIRECTION('',(0.,0.,1.));
#30443=DIRECTION('center_axis',(-1.,0.,0.));
#30444=DIRECTION('ref_axis',(0.,-1.,0.));
#30445=DIRECTION('',(0.,-1.,0.));
#30446=DIRECTION('',(0.,0.,1.));
#30447=DIRECTION('center_axis',(0.,-1.,0.));
#30448=DIRECTION('ref_axis',(1.,0.,0.));
#30449=DIRECTION('',(1.,0.,0.));
#30450=DIRECTION('',(0.,0.,1.));
#30451=DIRECTION('center_axis',(1.,0.,0.));
#30452=DIRECTION('ref_axis',(0.,1.,0.));
#30453=DIRECTION('',(0.,1.,0.));
#30454=DIRECTION('',(0.,0.,1.));
#30455=DIRECTION('center_axis',(0.72176022809836,-0.692143173870409,0.));
#30456=DIRECTION('ref_axis',(0.692143173870409,0.72176022809836,0.));
#30457=DIRECTION('',(0.692143173870409,0.72176022809836,0.));
#30458=DIRECTION('',(0.,0.,1.));
#30459=DIRECTION('center_axis',(0.,0.,1.));
#30460=DIRECTION('ref_axis',(-1.,0.,0.));
#30461=DIRECTION('center_axis',(0.,0.,1.));
#30462=DIRECTION('ref_axis',(-1.,0.,0.));
#30463=DIRECTION('',(0.,0.,1.));
#30464=DIRECTION('center_axis',(-1.,0.,0.));
#30465=DIRECTION('ref_axis',(0.,-1.,0.));
#30466=DIRECTION('',(0.,-1.,0.));
#30467=DIRECTION('center_axis',(0.,0.,1.));
#30468=DIRECTION('ref_axis',(1.,0.,0.));
#36135=CARTESIAN_POINT('',(0.,0.,0.));
#36136=CARTESIAN_POINT('Origin',(5.55111512312578E-16,19.8980255661466,
-22.));
#36137=CARTESIAN_POINT('',(0.476000000000002,18.7185,-22.));
#36138=CARTESIAN_POINT('',(0.476000000000002,20.4115,-22.));
#36139=CARTESIAN_POINT('',(0.476000000000002,20.4115,-22.));
#36140=CARTESIAN_POINT('',(0.273,20.6145,-22.));
#36141=CARTESIAN_POINT('Origin',(0.273,20.4115,-22.));
#36142=CARTESIAN_POINT('',(-0.273,20.6145,-22.));
#36143=CARTESIAN_POINT('',(0.273,20.6145,-22.));
#36144=CARTESIAN_POINT('',(-0.476000000000002,20.4115,-22.));
#36145=CARTESIAN_POINT('Origin',(-0.273,20.4115,-22.));
#36146=CARTESIAN_POINT('',(-0.475999999999999,18.7185,-22.));
#36147=CARTESIAN_POINT('',(-0.476000000000002,20.4115,-22.));
#36148=CARTESIAN_POINT('',(-0.749759876267637,18.6084492353546,-22.));
#36149=CARTESIAN_POINT('Origin',(-0.634999999999998,18.7185,-22.));
#36150=CARTESIAN_POINT('',(-1.55887524652215,19.4521869420016,-22.));
#36151=CARTESIAN_POINT('',(-0.749759876267637,18.6084492353546,-22.));
#36152=CARTESIAN_POINT('',(-1.55887524652215,19.9211869420016,-22.));
#36153=CARTESIAN_POINT('',(-1.55887524652215,19.4521869420016,-22.));
#36154=CARTESIAN_POINT('',(-3.19087524652215,19.9211869420016,-22.));
#36155=CARTESIAN_POINT('',(-1.55887524652215,19.9211869420016,-22.));
#36156=CARTESIAN_POINT('',(-3.19087524652215,18.3251869420016,-22.));
#36157=CARTESIAN_POINT('',(-3.19087524652215,19.9211869420016,-22.));
#36158=CARTESIAN_POINT('',(-4.34687524652215,18.3251869420016,-22.));
#36159=CARTESIAN_POINT('',(-3.19087524652215,18.3251869420016,-22.));
#36160=CARTESIAN_POINT('',(-4.34687524652215,20.1981869420016,-22.));
#36161=CARTESIAN_POINT('',(-4.34687524652215,18.3251869420016,-22.));
#36162=CARTESIAN_POINT('',(-4.06833369817656,20.5651518799515,-22.));
#36163=CARTESIAN_POINT('Origin',(-3.96587524652215,20.1981869420016,-22.));
#36164=CARTESIAN_POINT('',(-1.15958274644764,21.3772897382096,-22.));
#36165=CARTESIAN_POINT('',(-4.06833369817656,20.5651518799515,-22.));
#36166=CARTESIAN_POINT('',(-0.476500000000001,21.4708641902917,-22.));
#36167=CARTESIAN_POINT('Origin',(-0.476499999999996,18.9308641902917,-22.));
#36168=CARTESIAN_POINT('',(0.476499999999998,21.4708641902917,-22.));
#36169=CARTESIAN_POINT('',(0.476499999999999,21.4708641902917,-22.));
#36170=CARTESIAN_POINT('',(1.15958274644764,21.3772897382096,-22.));
#36171=CARTESIAN_POINT('Origin',(0.476499999999999,18.9308641902917,-22.));
#36172=CARTESIAN_POINT('',(4.06833369817657,20.5651518799515,-22.));
#36173=CARTESIAN_POINT('',(4.06833369817657,20.5651518799515,-22.));
#36174=CARTESIAN_POINT('',(4.34687524652215,20.1981869420016,-22.));
#36175=CARTESIAN_POINT('Origin',(3.96587524652215,20.1981869420016,-22.));
#36176=CARTESIAN_POINT('',(4.34687524652215,18.3251869420016,-22.));
#36177=CARTESIAN_POINT('',(4.34687524652215,18.3251869420016,-22.));
#36178=CARTESIAN_POINT('',(3.19087524652215,18.3251869420016,-22.));
#36179=CARTESIAN_POINT('',(3.19087524652215,18.3251869420016,-22.));
#36180=CARTESIAN_POINT('',(3.19087524652215,19.9211869420016,-22.));
#36181=CARTESIAN_POINT('',(3.19087524652215,19.9211869420016,-22.));
#36182=CARTESIAN_POINT('',(1.55887524652215,19.9211869420016,-22.));
#36183=CARTESIAN_POINT('',(1.55887524652215,19.9211869420016,-22.));
#36184=CARTESIAN_POINT('',(1.55887524652215,19.4521869420016,-22.));
#36185=CARTESIAN_POINT('',(1.55887524652215,19.4521869420016,-22.));
#36186=CARTESIAN_POINT('',(0.749759876267641,18.6084492353546,-22.));
#36187=CARTESIAN_POINT('',(0.749759876267641,18.6084492353546,-22.));
#36188=CARTESIAN_POINT('Origin',(0.635000000000002,18.7185,-22.));
#36189=CARTESIAN_POINT('Origin',(0.273,20.4115,0.));
#36190=CARTESIAN_POINT('',(0.476000000000002,20.4115,422.));
#36191=CARTESIAN_POINT('',(0.476000000000002,20.4115,0.));
#36192=CARTESIAN_POINT('',(0.273,20.6145,422.));
#36193=CARTESIAN_POINT('Origin',(0.273,20.4115,422.));
#36194=CARTESIAN_POINT('',(0.273,20.6145,0.));
#36195=CARTESIAN_POINT('Origin',(-0.273,20.6145,0.));
#36196=CARTESIAN_POINT('',(-0.273,20.6145,422.));
#36197=CARTESIAN_POINT('',(0.273,20.6145,422.));
#36198=CARTESIAN_POINT('',(-0.273,20.6145,0.));
#36199=CARTESIAN_POINT('Origin',(-0.273,20.4115,0.));
#36200=CARTESIAN_POINT('',(-0.476000000000002,20.4115,422.));
#36201=CARTESIAN_POINT('Origin',(-0.273,20.4115,422.));
#36202=CARTESIAN_POINT('',(-0.476000000000002,20.4115,0.));
#36203=CARTESIAN_POINT('Origin',(-0.475999999999999,18.7185,0.));
#36204=CARTESIAN_POINT('',(-0.475999999999999,18.7185,422.));
#36205=CARTESIAN_POINT('',(-0.476000000000002,20.4115,422.));
#36206=CARTESIAN_POINT('',(-0.475999999999999,18.7185,0.));
#36207=CARTESIAN_POINT('Origin',(-0.634999999999998,18.7185,0.));
#36208=CARTESIAN_POINT('',(-0.749759876267637,18.6084492353546,422.));
#36209=CARTESIAN_POINT('Origin',(-0.634999999999998,18.7185,422.));
#36210=CARTESIAN_POINT('',(-0.749759876267637,18.6084492353546,0.));
#36211=CARTESIAN_POINT('Origin',(-1.55887524652215,19.4521869420016,0.));
#36212=CARTESIAN_POINT('',(-1.55887524652215,19.4521869420016,422.));
#36213=CARTESIAN_POINT('',(-0.749759876267637,18.6084492353546,422.));
#36214=CARTESIAN_POINT('',(-1.55887524652215,19.4521869420016,0.));
#36215=CARTESIAN_POINT('Origin',(-1.55887524652215,19.9211869420016,0.));
#36216=CARTESIAN_POINT('',(-1.55887524652215,19.9211869420016,422.));
#36217=CARTESIAN_POINT('',(-1.55887524652215,19.4521869420016,422.));
#36218=CARTESIAN_POINT('',(-1.55887524652215,19.9211869420016,0.));
#36219=CARTESIAN_POINT('Origin',(-3.19087524652215,19.9211869420016,0.));
#36220=CARTESIAN_POINT('',(-3.19087524652215,19.9211869420016,422.));
#36221=CARTESIAN_POINT('',(-1.55887524652215,19.9211869420016,422.));
#36222=CARTESIAN_POINT('',(-3.19087524652215,19.9211869420016,0.));
#36223=CARTESIAN_POINT('Origin',(-3.19087524652215,18.3251869420016,0.));
#36224=CARTESIAN_POINT('',(-3.19087524652215,18.3251869420016,422.));
#36225=CARTESIAN_POINT('',(-3.19087524652215,19.9211869420016,422.));
#36226=CARTESIAN_POINT('',(-3.19087524652215,18.3251869420016,0.));
#36227=CARTESIAN_POINT('Origin',(-4.34687524652215,18.3251869420016,0.));
#36228=CARTESIAN_POINT('',(-4.34687524652215,18.3251869420016,422.));
#36229=CARTESIAN_POINT('',(-3.19087524652215,18.3251869420016,422.));
#36230=CARTESIAN_POINT('',(-4.34687524652215,18.3251869420016,0.));
#36231=CARTESIAN_POINT('Origin',(-4.34687524652215,20.1981869420016,0.));
#36232=CARTESIAN_POINT('',(-4.34687524652215,20.1981869420016,422.));
#36233=CARTESIAN_POINT('',(-4.34687524652215,18.3251869420016,422.));
#36234=CARTESIAN_POINT('',(-4.34687524652215,20.1981869420016,0.));
#36235=CARTESIAN_POINT('Origin',(-3.96587524652215,20.1981869420016,0.));
#36236=CARTESIAN_POINT('',(-4.06833369817656,20.5651518799515,422.));
#36237=CARTESIAN_POINT('Origin',(-3.96587524652215,20.1981869420016,422.));
#36238=CARTESIAN_POINT('',(-4.06833369817656,20.5651518799515,0.));
#36239=CARTESIAN_POINT('Origin',(-1.15958274644764,21.3772897382096,0.));
#36240=CARTESIAN_POINT('',(-1.15958274644764,21.3772897382096,422.));
#36241=CARTESIAN_POINT('',(-4.06833369817656,20.5651518799515,422.));
#36242=CARTESIAN_POINT('',(-1.15958274644764,21.3772897382096,0.));
#36243=CARTESIAN_POINT('Origin',(-0.476499999999996,18.9308641902917,0.));
#36244=CARTESIAN_POINT('',(-0.476500000000001,21.4708641902917,422.));
#36245=CARTESIAN_POINT('Origin',(-0.476499999999996,18.9308641902917,422.));
#36246=CARTESIAN_POINT('',(-0.476500000000001,21.4708641902917,0.));
#36247=CARTESIAN_POINT('Origin',(0.476499999999998,21.4708641902917,0.));
#36248=CARTESIAN_POINT('',(0.476499999999998,21.4708641902917,422.));
#36249=CARTESIAN_POINT('',(0.476499999999999,21.4708641902917,422.));
#36250=CARTESIAN_POINT('',(0.476499999999998,21.4708641902917,0.));
#36251=CARTESIAN_POINT('Origin',(0.476499999999999,18.9308641902917,0.));
#36252=CARTESIAN_POINT('',(1.15958274644764,21.3772897382096,422.));
#36253=CARTESIAN_POINT('Origin',(0.476499999999999,18.9308641902917,422.));
#36254=CARTESIAN_POINT('',(1.15958274644764,21.3772897382096,0.));
#36255=CARTESIAN_POINT('Origin',(4.06833369817657,20.5651518799515,0.));
#36256=CARTESIAN_POINT('',(4.06833369817657,20.5651518799515,422.));
#36257=CARTESIAN_POINT('',(4.06833369817657,20.5651518799515,422.));
#36258=CARTESIAN_POINT('',(4.06833369817657,20.5651518799515,0.));
#36259=CARTESIAN_POINT('Origin',(3.96587524652215,20.1981869420016,0.));
#36260=CARTESIAN_POINT('',(4.34687524652215,20.1981869420016,422.));
#36261=CARTESIAN_POINT('Origin',(3.96587524652215,20.1981869420016,422.));
#36262=CARTESIAN_POINT('',(4.34687524652215,20.1981869420016,0.));
#36263=CARTESIAN_POINT('Origin',(4.34687524652215,18.3251869420016,0.));
#36264=CARTESIAN_POINT('',(4.34687524652215,18.3251869420016,422.));
#36265=CARTESIAN_POINT('',(4.34687524652215,18.3251869420016,422.));
#36266=CARTESIAN_POINT('',(4.34687524652215,18.3251869420016,0.));
#36267=CARTESIAN_POINT('Origin',(3.19087524652215,18.3251869420016,0.));
#36268=CARTESIAN_POINT('',(3.19087524652215,18.3251869420016,422.));
#36269=CARTESIAN_POINT('',(3.19087524652215,18.3251869420016,422.));
#36270=CARTESIAN_POINT('',(3.19087524652215,18.3251869420016,0.));
#36271=CARTESIAN_POINT('Origin',(3.19087524652215,19.9211869420016,0.));
#36272=CARTESIAN_POINT('',(3.19087524652215,19.9211869420016,422.));
#36273=CARTESIAN_POINT('',(3.19087524652215,19.9211869420016,422.));
#36274=CARTESIAN_POINT('',(3.19087524652215,19.9211869420016,0.));
#36275=CARTESIAN_POINT('Origin',(1.55887524652215,19.9211869420016,0.));
#36276=CARTESIAN_POINT('',(1.55887524652215,19.9211869420016,422.));
#36277=CARTESIAN_POINT('',(1.55887524652215,19.9211869420016,422.));
#36278=CARTESIAN_POINT('',(1.55887524652215,19.9211869420016,0.));
#36279=CARTESIAN_POINT('Origin',(1.55887524652215,19.4521869420016,0.));
#36280=CARTESIAN_POINT('',(1.55887524652215,19.4521869420016,422.));
#36281=CARTESIAN_POINT('',(1.55887524652215,19.4521869420016,422.));
#36282=CARTESIAN_POINT('',(1.55887524652215,19.4521869420016,0.));
#36283=CARTESIAN_POINT('Origin',(0.749759876267641,18.6084492353546,0.));
#36284=CARTESIAN_POINT('',(0.749759876267641,18.6084492353546,422.));
#36285=CARTESIAN_POINT('',(0.749759876267641,18.6084492353546,422.));
#36286=CARTESIAN_POINT('',(0.749759876267641,18.6084492353546,0.));
#36287=CARTESIAN_POINT('Origin',(0.635000000000002,18.7185,0.));
#36288=CARTESIAN_POINT('',(0.476000000000002,18.7185,422.));
#36289=CARTESIAN_POINT('Origin',(0.635000000000002,18.7185,422.));
#36290=CARTESIAN_POINT('',(0.476000000000002,18.7185,0.));
#36291=CARTESIAN_POINT('Origin',(0.476000000000002,20.4115,0.));
#36292=CARTESIAN_POINT('',(0.476000000000002,20.4115,422.));
#36293=CARTESIAN_POINT('Origin',(5.55111512312578E-16,19.8980255661466,
422.));
#215590=UNCERTAINTY_MEASURE_WITH_UNIT(LENGTH_MEASURE(0.01),#215610,
'DISTANCE_ACCURACY_VALUE',
'Maximum model space distance between geometric entities at asserted c
onnectivities');
#215598=UNCERTAINTY_MEASURE_WITH_UNIT(LENGTH_MEASURE(0.01),#215610,
'DISTANCE_ACCURACY_VALUE',
'Maximum model space distance between geometric entities at asserted c
onnectivities');
#215601=(
GEOMETRIC_REPRESENTATION_CONTEXT(3)
GLOBAL_UNCERTAINTY_ASSIGNED_CONTEXT((#215590))
GLOBAL_UNIT_ASSIGNED_CONTEXT((#215610,#215612,#215613))
REPRESENTATION_CONTEXT('','3D')
);
#215609=(
GEOMETRIC_REPRESENTATION_CONTEXT(3)
GLOBAL_UNCERTAINTY_ASSIGNED_CONTEXT((#215598))
GLOBAL_UNIT_ASSIGNED_CONTEXT((#215610,#215612,#215613))
REPRESENTATION_CONTEXT('','3D')
);
#215610=(
LENGTH_UNIT()
NAMED_UNIT(*)
SI_UNIT(.MILLI.,.METRE.)
);
#215612=(
NAMED_UNIT(*)
PLANE_ANGLE_UNIT()
SI_UNIT($,.RADIAN.)
);
#215613=(
NAMED_UNIT(*)
SI_UNIT($,.STERADIAN.)
SOLID_ANGLE_UNIT()
);
#215616=SHAPE_DEFINITION_REPRESENTATION(#215626,#215645);
#215626=PRODUCT_DEFINITION_SHAPE('',$,#215656);
#215645=SHAPE_REPRESENTATION('',(#28227),#215601);
#215653=PRODUCT_DEFINITION_CONTEXT('part definition',#215685,'design');
#215656=PRODUCT_DEFINITION('2026-10-04-10-37-11-877','TopStripTop',#215666,
#215653);
#215666=PRODUCT_DEFINITION_FORMATION('',$,#215689);
#215685=APPLICATION_CONTEXT(
'Core Data for Automotive Mechanical Design Process');
#215686=PRODUCT_CONTEXT('part definition',#215685,'mechanical');
#215689=PRODUCT('2026-10-04-10-37-11-877','TopStripTop',$,(#215686));
#215698=PRESENTATION_STYLE_ASSIGNMENT((#215700));
#215700=SURFACE_STYLE_USAGE(.BOTH.,#215702);
#215702=SURFACE_SIDE_STYLE('',(#215704));
#215704=SURFACE_STYLE_FILL_AREA(#215706);
#215706=FILL_AREA_STYLE('Opaque(245,245,246)',(#215708));
#215708=FILL_AREA_STYLE_COLOUR('Opaque(245,245,246)',#215710);
#215710=COLOUR_RGB('Opaque(245,245,246)', 0.66274510, 0.83137255, 0.94901961);
ENDSEC;
END-ISO-10303-21;
